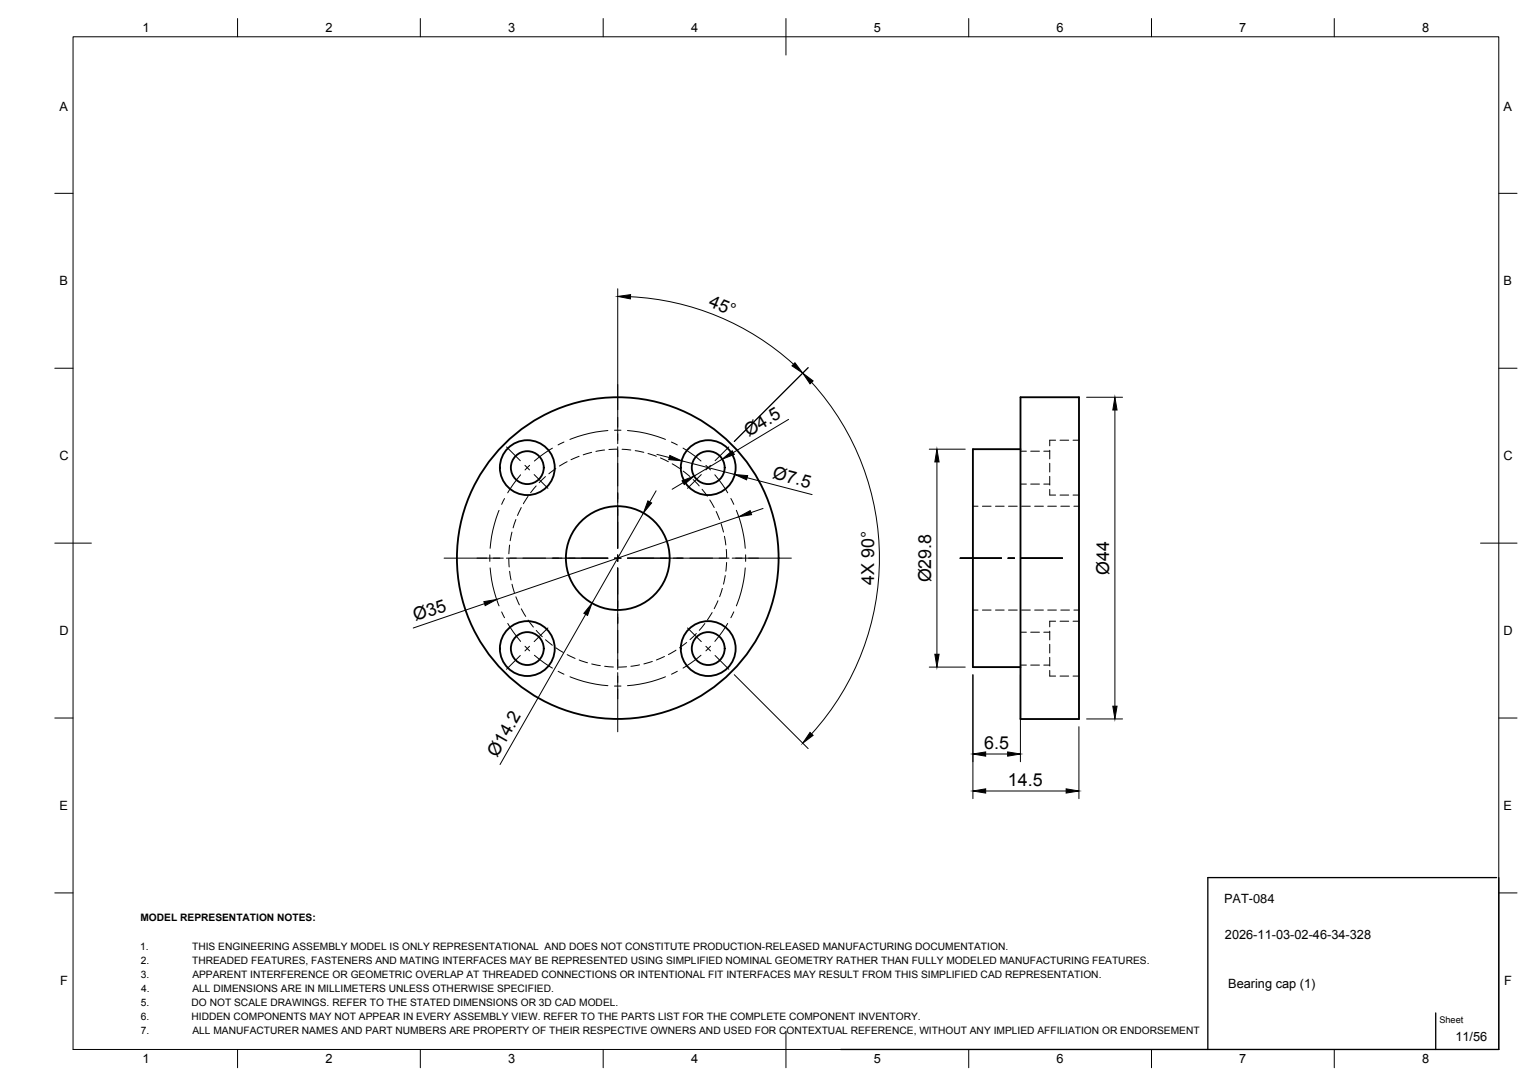
ISO-10303-21;
HEADER;
/* Generated by software containing ST-Developer
 * from STEP Tools, Inc. (www.steptools.com) 
 */

FILE_DESCRIPTION(
/* description */ ('Quick-return (Whitworth) mechanism'),
/* implementation_level */ '2;1');

FILE_NAME(
/* name */ 'Bearing cap (1).step',
/* time_stamp */ '2026-10-28T03:25:57-07:00',
/* author */ (''),
/* organization */ (''),
/* preprocessor_version */ 'ST-DEVELOPER v20.2',
/* originating_system */ 'Autodesk Translation Framework v15.17.0.0',
/* authorisation */ '');

FILE_SCHEMA (('AUTOMOTIVE_DESIGN { 1 0 10303 214 3 1 1 }'));
ENDSEC;

DATA;
#10=MECHANICAL_DESIGN_GEOMETRIC_PRESENTATION_REPRESENTATION('',(#496),#14878);
#408=SHAPE_REPRESENTATION_RELATIONSHIP('SRR','None',#15076,#452);
#452=ADVANCED_BREP_SHAPE_REPRESENTATION('',(#548),#14833);
#496=STYLED_ITEM('',(#15406),#548);
#548=MANIFOLD_SOLID_BREP('Body1',#7850);
#666=FACE_BOUND('',#1696,.T.);
#667=FACE_BOUND('',#1699,.T.);
#668=FACE_BOUND('',#1702,.T.);
#669=FACE_BOUND('',#1705,.T.);
#670=FACE_BOUND('',#1712,.T.);
#671=FACE_BOUND('',#1716,.T.);
#672=FACE_BOUND('',#1717,.T.);
#673=FACE_BOUND('',#1718,.T.);
#674=FACE_BOUND('',#1719,.T.);
#675=FACE_BOUND('',#1720,.T.);
#676=FACE_BOUND('',#1722,.T.);
#677=FACE_BOUND('',#1723,.T.);
#678=FACE_BOUND('',#1724,.T.);
#679=FACE_BOUND('',#1725,.T.);
#680=FACE_BOUND('',#1726,.T.);
#831=PLANE('',#8628);
#832=PLANE('',#8633);
#833=PLANE('',#8638);
#834=PLANE('',#8643);
#835=PLANE('',#8656);
#836=PLANE('',#8663);
#837=PLANE('',#8664);
#1153=FACE_OUTER_BOUND('',#1694,.T.);
#1154=FACE_OUTER_BOUND('',#1695,.T.);
#1155=FACE_OUTER_BOUND('',#1697,.T.);
#1156=FACE_OUTER_BOUND('',#1698,.T.);
#1157=FACE_OUTER_BOUND('',#1700,.T.);
#1158=FACE_OUTER_BOUND('',#1701,.T.);
#1159=FACE_OUTER_BOUND('',#1703,.T.);
#1160=FACE_OUTER_BOUND('',#1704,.T.);
#1161=FACE_OUTER_BOUND('',#1706,.T.);
#1162=FACE_OUTER_BOUND('',#1707,.T.);
#1163=FACE_OUTER_BOUND('',#1708,.T.);
#1164=FACE_OUTER_BOUND('',#1709,.T.);
#1165=FACE_OUTER_BOUND('',#1710,.T.);
#1166=FACE_OUTER_BOUND('',#1711,.T.);
#1167=FACE_OUTER_BOUND('',#1713,.T.);
#1168=FACE_OUTER_BOUND('',#1714,.T.);
#1169=FACE_OUTER_BOUND('',#1715,.T.);
#1170=FACE_OUTER_BOUND('',#1721,.T.);
#1694=EDGE_LOOP('',(#5732,#5733,#5734,#5735));
#1695=EDGE_LOOP('',(#5736));
#1696=EDGE_LOOP('',(#5737));
#1697=EDGE_LOOP('',(#5738,#5739,#5740,#5741));
#1698=EDGE_LOOP('',(#5742));
#1699=EDGE_LOOP('',(#5743));
#1700=EDGE_LOOP('',(#5744,#5745,#5746,#5747));
#1701=EDGE_LOOP('',(#5748));
#1702=EDGE_LOOP('',(#5749));
#1703=EDGE_LOOP('',(#5750,#5751,#5752,#5753));
#1704=EDGE_LOOP('',(#5754));
#1705=EDGE_LOOP('',(#5755));
#1706=EDGE_LOOP('',(#5756,#5757,#5758,#5759));
#1707=EDGE_LOOP('',(#5760,#5761,#5762,#5763));
#1708=EDGE_LOOP('',(#5764,#5765,#5766,#5767));
#1709=EDGE_LOOP('',(#5768,#5769,#5770,#5771));
#1710=EDGE_LOOP('',(#5772,#5773,#5774,#5775));
#1711=EDGE_LOOP('',(#5776));
#1712=EDGE_LOOP('',(#5777));
#1713=EDGE_LOOP('',(#5778,#5779,#5780,#5781));
#1714=EDGE_LOOP('',(#5782,#5783,#5784,#5785));
#1715=EDGE_LOOP('',(#5786));
#1716=EDGE_LOOP('',(#5787));
#1717=EDGE_LOOP('',(#5788));
#1718=EDGE_LOOP('',(#5789));
#1719=EDGE_LOOP('',(#5790));
#1720=EDGE_LOOP('',(#5791));
#1721=EDGE_LOOP('',(#5792));
#1722=EDGE_LOOP('',(#5793));
#1723=EDGE_LOOP('',(#5794));
#1724=EDGE_LOOP('',(#5795));
#1725=EDGE_LOOP('',(#5796));
#1726=EDGE_LOOP('',(#5797));
#2271=LINE('',#12594,#2794);
#2272=LINE('',#12603,#2795);
#2273=LINE('',#12612,#2796);
#2274=LINE('',#12621,#2797);
#2275=LINE('',#12629,#2798);
#2276=LINE('',#12633,#2799);
#2277=LINE('',#12637,#2800);
#2278=LINE('',#12641,#2801);
#2279=LINE('',#12646,#2802);
#2280=LINE('',#12654,#2803);
#2281=LINE('',#12659,#2804);
#2794=VECTOR('',#9984,0.375);
#2795=VECTOR('',#9995,0.375);
#2796=VECTOR('',#10006,0.375);
#2797=VECTOR('',#10017,0.375);
#2798=VECTOR('',#10028,0.225);
#2799=VECTOR('',#10033,0.225);
#2800=VECTOR('',#10038,0.225);
#2801=VECTOR('',#10043,0.225);
#2802=VECTOR('',#10048,1.49);
#2803=VECTOR('',#10059,0.71);
#2804=VECTOR('',#10064,2.2);
#3342=CIRCLE('',#8626,0.375);
#3343=CIRCLE('',#8627,0.375);
#3344=CIRCLE('',#8629,0.225);
#3345=CIRCLE('',#8631,0.375);
#3346=CIRCLE('',#8632,0.375);
#3347=CIRCLE('',#8634,0.225);
#3348=CIRCLE('',#8636,0.375);
#3349=CIRCLE('',#8637,0.375);
#3350=CIRCLE('',#8639,0.225);
#3351=CIRCLE('',#8641,0.375);
#3352=CIRCLE('',#8642,0.375);
#3353=CIRCLE('',#8644,0.225);
#3354=CIRCLE('',#8646,0.225);
#3355=CIRCLE('',#8648,0.225);
#3356=CIRCLE('',#8650,0.225);
#3357=CIRCLE('',#8652,0.225);
#3358=CIRCLE('',#8654,1.49);
#3359=CIRCLE('',#8655,1.49);
#3360=CIRCLE('',#8657,0.71);
#3361=CIRCLE('',#8659,0.71);
#3362=CIRCLE('',#8661,2.2);
#3363=CIRCLE('',#8662,2.2);
#3789=VERTEX_POINT('',#12591);
#3790=VERTEX_POINT('',#12593);
#3791=VERTEX_POINT('',#12597);
#3792=VERTEX_POINT('',#12600);
#3793=VERTEX_POINT('',#12602);
#3794=VERTEX_POINT('',#12606);
#3795=VERTEX_POINT('',#12609);
#3796=VERTEX_POINT('',#12611);
#3797=VERTEX_POINT('',#12615);
#3798=VERTEX_POINT('',#12618);
#3799=VERTEX_POINT('',#12620);
#3800=VERTEX_POINT('',#12624);
#3801=VERTEX_POINT('',#12627);
#3802=VERTEX_POINT('',#12631);
#3803=VERTEX_POINT('',#12635);
#3804=VERTEX_POINT('',#12639);
#3805=VERTEX_POINT('',#12643);
#3806=VERTEX_POINT('',#12645);
#3807=VERTEX_POINT('',#12649);
#3808=VERTEX_POINT('',#12652);
#3809=VERTEX_POINT('',#12656);
#3810=VERTEX_POINT('',#12658);
#4523=EDGE_CURVE('',#3789,#3789,#3342,.T.);
#4524=EDGE_CURVE('',#3789,#3790,#2271,.T.);
#4525=EDGE_CURVE('',#3790,#3790,#3343,.T.);
#4526=EDGE_CURVE('',#3791,#3791,#3344,.T.);
#4527=EDGE_CURVE('',#3792,#3792,#3345,.T.);
#4528=EDGE_CURVE('',#3792,#3793,#2272,.T.);
#4529=EDGE_CURVE('',#3793,#3793,#3346,.T.);
#4530=EDGE_CURVE('',#3794,#3794,#3347,.T.);
#4531=EDGE_CURVE('',#3795,#3795,#3348,.T.);
#4532=EDGE_CURVE('',#3795,#3796,#2273,.T.);
#4533=EDGE_CURVE('',#3796,#3796,#3349,.T.);
#4534=EDGE_CURVE('',#3797,#3797,#3350,.T.);
#4535=EDGE_CURVE('',#3798,#3798,#3351,.T.);
#4536=EDGE_CURVE('',#3798,#3799,#2274,.T.);
#4537=EDGE_CURVE('',#3799,#3799,#3352,.T.);
#4538=EDGE_CURVE('',#3800,#3800,#3353,.T.);
#4539=EDGE_CURVE('',#3801,#3801,#3354,.T.);
#4540=EDGE_CURVE('',#3801,#3791,#2275,.T.);
#4541=EDGE_CURVE('',#3802,#3802,#3355,.T.);
#4542=EDGE_CURVE('',#3802,#3794,#2276,.T.);
#4543=EDGE_CURVE('',#3803,#3803,#3356,.T.);
#4544=EDGE_CURVE('',#3803,#3797,#2277,.T.);
#4545=EDGE_CURVE('',#3804,#3804,#3357,.T.);
#4546=EDGE_CURVE('',#3804,#3800,#2278,.T.);
#4547=EDGE_CURVE('',#3805,#3805,#3358,.T.);
#4548=EDGE_CURVE('',#3805,#3806,#2279,.T.);
#4549=EDGE_CURVE('',#3806,#3806,#3359,.T.);
#4550=EDGE_CURVE('',#3807,#3807,#3360,.T.);
#4551=EDGE_CURVE('',#3808,#3808,#3361,.T.);
#4552=EDGE_CURVE('',#3808,#3807,#2280,.T.);
#4553=EDGE_CURVE('',#3809,#3809,#3362,.T.);
#4554=EDGE_CURVE('',#3809,#3810,#2281,.T.);
#4555=EDGE_CURVE('',#3810,#3810,#3363,.T.);
#5732=ORIENTED_EDGE('',*,*,#4523,.F.);
#5733=ORIENTED_EDGE('',*,*,#4524,.T.);
#5734=ORIENTED_EDGE('',*,*,#4525,.F.);
#5735=ORIENTED_EDGE('',*,*,#4524,.F.);
#5736=ORIENTED_EDGE('',*,*,#4523,.T.);
#5737=ORIENTED_EDGE('',*,*,#4526,.F.);
#5738=ORIENTED_EDGE('',*,*,#4527,.F.);
#5739=ORIENTED_EDGE('',*,*,#4528,.T.);
#5740=ORIENTED_EDGE('',*,*,#4529,.F.);
#5741=ORIENTED_EDGE('',*,*,#4528,.F.);
#5742=ORIENTED_EDGE('',*,*,#4527,.T.);
#5743=ORIENTED_EDGE('',*,*,#4530,.F.);
#5744=ORIENTED_EDGE('',*,*,#4531,.F.);
#5745=ORIENTED_EDGE('',*,*,#4532,.T.);
#5746=ORIENTED_EDGE('',*,*,#4533,.F.);
#5747=ORIENTED_EDGE('',*,*,#4532,.F.);
#5748=ORIENTED_EDGE('',*,*,#4531,.T.);
#5749=ORIENTED_EDGE('',*,*,#4534,.F.);
#5750=ORIENTED_EDGE('',*,*,#4535,.F.);
#5751=ORIENTED_EDGE('',*,*,#4536,.T.);
#5752=ORIENTED_EDGE('',*,*,#4537,.F.);
#5753=ORIENTED_EDGE('',*,*,#4536,.F.);
#5754=ORIENTED_EDGE('',*,*,#4535,.T.);
#5755=ORIENTED_EDGE('',*,*,#4538,.F.);
#5756=ORIENTED_EDGE('',*,*,#4539,.F.);
#5757=ORIENTED_EDGE('',*,*,#4540,.T.);
#5758=ORIENTED_EDGE('',*,*,#4526,.T.);
#5759=ORIENTED_EDGE('',*,*,#4540,.F.);
#5760=ORIENTED_EDGE('',*,*,#4541,.F.);
#5761=ORIENTED_EDGE('',*,*,#4542,.T.);
#5762=ORIENTED_EDGE('',*,*,#4530,.T.);
#5763=ORIENTED_EDGE('',*,*,#4542,.F.);
#5764=ORIENTED_EDGE('',*,*,#4543,.F.);
#5765=ORIENTED_EDGE('',*,*,#4544,.T.);
#5766=ORIENTED_EDGE('',*,*,#4534,.T.);
#5767=ORIENTED_EDGE('',*,*,#4544,.F.);
#5768=ORIENTED_EDGE('',*,*,#4545,.F.);
#5769=ORIENTED_EDGE('',*,*,#4546,.T.);
#5770=ORIENTED_EDGE('',*,*,#4538,.T.);
#5771=ORIENTED_EDGE('',*,*,#4546,.F.);
#5772=ORIENTED_EDGE('',*,*,#4547,.F.);
#5773=ORIENTED_EDGE('',*,*,#4548,.T.);
#5774=ORIENTED_EDGE('',*,*,#4549,.T.);
#5775=ORIENTED_EDGE('',*,*,#4548,.F.);
#5776=ORIENTED_EDGE('',*,*,#4549,.F.);
#5777=ORIENTED_EDGE('',*,*,#4550,.F.);
#5778=ORIENTED_EDGE('',*,*,#4551,.F.);
#5779=ORIENTED_EDGE('',*,*,#4552,.T.);
#5780=ORIENTED_EDGE('',*,*,#4550,.T.);
#5781=ORIENTED_EDGE('',*,*,#4552,.F.);
#5782=ORIENTED_EDGE('',*,*,#4553,.F.);
#5783=ORIENTED_EDGE('',*,*,#4554,.T.);
#5784=ORIENTED_EDGE('',*,*,#4555,.T.);
#5785=ORIENTED_EDGE('',*,*,#4554,.F.);
#5786=ORIENTED_EDGE('',*,*,#4553,.T.);
#5787=ORIENTED_EDGE('',*,*,#4551,.T.);
#5788=ORIENTED_EDGE('',*,*,#4537,.T.);
#5789=ORIENTED_EDGE('',*,*,#4533,.T.);
#5790=ORIENTED_EDGE('',*,*,#4529,.T.);
#5791=ORIENTED_EDGE('',*,*,#4525,.T.);
#5792=ORIENTED_EDGE('',*,*,#4555,.F.);
#5793=ORIENTED_EDGE('',*,*,#4547,.T.);
#5794=ORIENTED_EDGE('',*,*,#4545,.T.);
#5795=ORIENTED_EDGE('',*,*,#4543,.T.);
#5796=ORIENTED_EDGE('',*,*,#4541,.T.);
#5797=ORIENTED_EDGE('',*,*,#4539,.T.);
#7267=CYLINDRICAL_SURFACE('',#8625,0.375);
#7268=CYLINDRICAL_SURFACE('',#8630,0.375);
#7269=CYLINDRICAL_SURFACE('',#8635,0.375);
#7270=CYLINDRICAL_SURFACE('',#8640,0.375);
#7271=CYLINDRICAL_SURFACE('',#8645,0.225);
#7272=CYLINDRICAL_SURFACE('',#8647,0.225);
#7273=CYLINDRICAL_SURFACE('',#8649,0.225);
#7274=CYLINDRICAL_SURFACE('',#8651,0.225);
#7275=CYLINDRICAL_SURFACE('',#8653,1.49);
#7276=CYLINDRICAL_SURFACE('',#8658,0.71);
#7277=CYLINDRICAL_SURFACE('',#8660,2.2);
#7484=ADVANCED_FACE('',(#1153),#7267,.F.);
#7485=ADVANCED_FACE('',(#1154,#666),#831,.T.);
#7486=ADVANCED_FACE('',(#1155),#7268,.F.);
#7487=ADVANCED_FACE('',(#1156,#667),#832,.T.);
#7488=ADVANCED_FACE('',(#1157),#7269,.F.);
#7489=ADVANCED_FACE('',(#1158,#668),#833,.T.);
#7490=ADVANCED_FACE('',(#1159),#7270,.F.);
#7491=ADVANCED_FACE('',(#1160,#669),#834,.T.);
#7492=ADVANCED_FACE('',(#1161),#7271,.F.);
#7493=ADVANCED_FACE('',(#1162),#7272,.F.);
#7494=ADVANCED_FACE('',(#1163),#7273,.F.);
#7495=ADVANCED_FACE('',(#1164),#7274,.F.);
#7496=ADVANCED_FACE('',(#1165),#7275,.T.);
#7497=ADVANCED_FACE('',(#1166,#670),#835,.F.);
#7498=ADVANCED_FACE('',(#1167),#7276,.F.);
#7499=ADVANCED_FACE('',(#1168),#7277,.T.);
#7500=ADVANCED_FACE('',(#1169,#671,#672,#673,#674,#675),#836,.T.);
#7501=ADVANCED_FACE('',(#1170,#676,#677,#678,#679,#680),#837,.F.);
#7850=CLOSED_SHELL('',(#7484,#7485,#7486,#7487,#7488,#7489,#7490,#7491,
#7492,#7493,#7494,#7495,#7496,#7497,#7498,#7499,#7500,#7501));
#8624=AXIS2_PLACEMENT_3D('',#12589,#9978,#9979);
#8625=AXIS2_PLACEMENT_3D('',#12590,#9980,#9981);
#8626=AXIS2_PLACEMENT_3D('',#12592,#9982,#9983);
#8627=AXIS2_PLACEMENT_3D('',#12595,#9985,#9986);
#8628=AXIS2_PLACEMENT_3D('',#12596,#9987,#9988);
#8629=AXIS2_PLACEMENT_3D('',#12598,#9989,#9990);
#8630=AXIS2_PLACEMENT_3D('',#12599,#9991,#9992);
#8631=AXIS2_PLACEMENT_3D('',#12601,#9993,#9994);
#8632=AXIS2_PLACEMENT_3D('',#12604,#9996,#9997);
#8633=AXIS2_PLACEMENT_3D('',#12605,#9998,#9999);
#8634=AXIS2_PLACEMENT_3D('',#12607,#10000,#10001);
#8635=AXIS2_PLACEMENT_3D('',#12608,#10002,#10003);
#8636=AXIS2_PLACEMENT_3D('',#12610,#10004,#10005);
#8637=AXIS2_PLACEMENT_3D('',#12613,#10007,#10008);
#8638=AXIS2_PLACEMENT_3D('',#12614,#10009,#10010);
#8639=AXIS2_PLACEMENT_3D('',#12616,#10011,#10012);
#8640=AXIS2_PLACEMENT_3D('',#12617,#10013,#10014);
#8641=AXIS2_PLACEMENT_3D('',#12619,#10015,#10016);
#8642=AXIS2_PLACEMENT_3D('',#12622,#10018,#10019);
#8643=AXIS2_PLACEMENT_3D('',#12623,#10020,#10021);
#8644=AXIS2_PLACEMENT_3D('',#12625,#10022,#10023);
#8645=AXIS2_PLACEMENT_3D('',#12626,#10024,#10025);
#8646=AXIS2_PLACEMENT_3D('',#12628,#10026,#10027);
#8647=AXIS2_PLACEMENT_3D('',#12630,#10029,#10030);
#8648=AXIS2_PLACEMENT_3D('',#12632,#10031,#10032);
#8649=AXIS2_PLACEMENT_3D('',#12634,#10034,#10035);
#8650=AXIS2_PLACEMENT_3D('',#12636,#10036,#10037);
#8651=AXIS2_PLACEMENT_3D('',#12638,#10039,#10040);
#8652=AXIS2_PLACEMENT_3D('',#12640,#10041,#10042);
#8653=AXIS2_PLACEMENT_3D('',#12642,#10044,#10045);
#8654=AXIS2_PLACEMENT_3D('',#12644,#10046,#10047);
#8655=AXIS2_PLACEMENT_3D('',#12647,#10049,#10050);
#8656=AXIS2_PLACEMENT_3D('',#12648,#10051,#10052);
#8657=AXIS2_PLACEMENT_3D('',#12650,#10053,#10054);
#8658=AXIS2_PLACEMENT_3D('',#12651,#10055,#10056);
#8659=AXIS2_PLACEMENT_3D('',#12653,#10057,#10058);
#8660=AXIS2_PLACEMENT_3D('',#12655,#10060,#10061);
#8661=AXIS2_PLACEMENT_3D('',#12657,#10062,#10063);
#8662=AXIS2_PLACEMENT_3D('',#12660,#10065,#10066);
#8663=AXIS2_PLACEMENT_3D('',#12661,#10067,#10068);
#8664=AXIS2_PLACEMENT_3D('',#12662,#10069,#10070);
#9978=DIRECTION('axis',(0.,0.,1.));
#9979=DIRECTION('refdir',(1.,0.,0.));
#9980=DIRECTION('center_axis',(0.,0.,1.));
#9981=DIRECTION('ref_axis',(1.,0.,0.));
#9982=DIRECTION('center_axis',(0.,0.,1.));
#9983=DIRECTION('ref_axis',(1.,0.,0.));
#9984=DIRECTION('',(0.,0.,1.));
#9985=DIRECTION('center_axis',(0.,0.,-1.));
#9986=DIRECTION('ref_axis',(1.,0.,0.));
#9987=DIRECTION('center_axis',(0.,0.,1.));
#9988=DIRECTION('ref_axis',(1.,0.,0.));
#9989=DIRECTION('center_axis',(0.,0.,1.));
#9990=DIRECTION('ref_axis',(1.,0.,0.));
#9991=DIRECTION('center_axis',(0.,0.,1.));
#9992=DIRECTION('ref_axis',(1.,0.,0.));
#9993=DIRECTION('center_axis',(0.,0.,1.));
#9994=DIRECTION('ref_axis',(1.,0.,0.));
#9995=DIRECTION('',(0.,0.,1.));
#9996=DIRECTION('center_axis',(0.,0.,-1.));
#9997=DIRECTION('ref_axis',(1.,0.,0.));
#9998=DIRECTION('center_axis',(0.,0.,1.));
#9999=DIRECTION('ref_axis',(1.,0.,0.));
#10000=DIRECTION('center_axis',(0.,0.,1.));
#10001=DIRECTION('ref_axis',(1.,0.,0.));
#10002=DIRECTION('center_axis',(0.,0.,1.));
#10003=DIRECTION('ref_axis',(1.,0.,0.));
#10004=DIRECTION('center_axis',(0.,0.,1.));
#10005=DIRECTION('ref_axis',(1.,0.,0.));
#10006=DIRECTION('',(0.,0.,1.));
#10007=DIRECTION('center_axis',(0.,0.,-1.));
#10008=DIRECTION('ref_axis',(1.,0.,0.));
#10009=DIRECTION('center_axis',(0.,0.,1.));
#10010=DIRECTION('ref_axis',(1.,0.,0.));
#10011=DIRECTION('center_axis',(0.,0.,1.));
#10012=DIRECTION('ref_axis',(1.,0.,0.));
#10013=DIRECTION('center_axis',(0.,0.,1.));
#10014=DIRECTION('ref_axis',(1.,0.,0.));
#10015=DIRECTION('center_axis',(0.,0.,1.));
#10016=DIRECTION('ref_axis',(1.,0.,0.));
#10017=DIRECTION('',(0.,0.,1.));
#10018=DIRECTION('center_axis',(0.,0.,-1.));
#10019=DIRECTION('ref_axis',(1.,0.,0.));
#10020=DIRECTION('center_axis',(0.,0.,1.));
#10021=DIRECTION('ref_axis',(1.,0.,0.));
#10022=DIRECTION('center_axis',(0.,0.,1.));
#10023=DIRECTION('ref_axis',(1.,0.,0.));
#10024=DIRECTION('center_axis',(0.,0.,1.));
#10025=DIRECTION('ref_axis',(1.,0.,0.));
#10026=DIRECTION('center_axis',(0.,0.,1.));
#10027=DIRECTION('ref_axis',(1.,0.,0.));
#10028=DIRECTION('',(0.,0.,1.));
#10029=DIRECTION('center_axis',(0.,0.,1.));
#10030=DIRECTION('ref_axis',(1.,0.,0.));
#10031=DIRECTION('center_axis',(0.,0.,1.));
#10032=DIRECTION('ref_axis',(1.,0.,0.));
#10033=DIRECTION('',(0.,0.,1.));
#10034=DIRECTION('center_axis',(0.,0.,1.));
#10035=DIRECTION('ref_axis',(1.,0.,0.));
#10036=DIRECTION('center_axis',(0.,0.,1.));
#10037=DIRECTION('ref_axis',(1.,0.,0.));
#10038=DIRECTION('',(0.,0.,1.));
#10039=DIRECTION('center_axis',(0.,0.,1.));
#10040=DIRECTION('ref_axis',(1.,0.,0.));
#10041=DIRECTION('center_axis',(0.,0.,1.));
#10042=DIRECTION('ref_axis',(1.,0.,0.));
#10043=DIRECTION('',(0.,0.,1.));
#10044=DIRECTION('center_axis',(0.,0.,1.));
#10045=DIRECTION('ref_axis',(1.,0.,0.));
#10046=DIRECTION('center_axis',(0.,0.,1.));
#10047=DIRECTION('ref_axis',(1.,0.,0.));
#10048=DIRECTION('',(0.,0.,-1.));
#10049=DIRECTION('center_axis',(0.,0.,1.));
#10050=DIRECTION('ref_axis',(1.,0.,0.));
#10051=DIRECTION('center_axis',(0.,0.,1.));
#10052=DIRECTION('ref_axis',(1.,0.,0.));
#10053=DIRECTION('center_axis',(0.,0.,-1.));
#10054=DIRECTION('ref_axis',(1.,0.,0.));
#10055=DIRECTION('center_axis',(0.,0.,1.));
#10056=DIRECTION('ref_axis',(1.,0.,0.));
#10057=DIRECTION('center_axis',(0.,0.,-1.));
#10058=DIRECTION('ref_axis',(1.,0.,0.));
#10059=DIRECTION('',(0.,0.,-1.));
#10060=DIRECTION('center_axis',(0.,0.,1.));
#10061=DIRECTION('ref_axis',(1.,0.,0.));
#10062=DIRECTION('center_axis',(0.,0.,1.));
#10063=DIRECTION('ref_axis',(1.,0.,0.));
#10064=DIRECTION('',(0.,0.,-1.));
#10065=DIRECTION('center_axis',(0.,0.,1.));
#10066=DIRECTION('ref_axis',(1.,0.,0.));
#10067=DIRECTION('center_axis',(0.,0.,1.));
#10068=DIRECTION('ref_axis',(1.,0.,0.));
#10069=DIRECTION('center_axis',(0.,0.,1.));
#10070=DIRECTION('ref_axis',(1.,0.,0.));
#12589=CARTESIAN_POINT('',(0.,0.,0.));
#12590=CARTESIAN_POINT('Origin',(-1.23743686707646,4.76256313292354,4.));
#12591=CARTESIAN_POINT('',(-1.61243686707646,4.76256313292354,4.));
#12592=CARTESIAN_POINT('Origin',(-1.23743686707646,4.76256313292354,4.));
#12593=CARTESIAN_POINT('',(-1.61243686707646,4.76256313292354,4.4));
#12594=CARTESIAN_POINT('',(-1.61243686707646,4.76256313292354,4.));
#12595=CARTESIAN_POINT('Origin',(-1.23743686707646,4.76256313292354,4.4));
#12596=CARTESIAN_POINT('Origin',(-1.23743686707646,4.76256313292354,4.));
#12597=CARTESIAN_POINT('',(-1.46243686707646,4.76256313292354,4.));
#12598=CARTESIAN_POINT('Origin',(-1.23743686707646,4.76256313292354,4.));
#12599=CARTESIAN_POINT('Origin',(-1.23743686707646,7.23743686707646,4.));
#12600=CARTESIAN_POINT('',(-1.61243686707646,7.23743686707646,4.));
#12601=CARTESIAN_POINT('Origin',(-1.23743686707646,7.23743686707646,4.));
#12602=CARTESIAN_POINT('',(-1.61243686707646,7.23743686707646,4.4));
#12603=CARTESIAN_POINT('',(-1.61243686707646,7.23743686707646,4.));
#12604=CARTESIAN_POINT('Origin',(-1.23743686707646,7.23743686707646,4.4));
#12605=CARTESIAN_POINT('Origin',(-1.23743686707646,7.23743686707646,4.));
#12606=CARTESIAN_POINT('',(-1.46243686707646,7.23743686707646,4.));
#12607=CARTESIAN_POINT('Origin',(-1.23743686707646,7.23743686707646,4.));
#12608=CARTESIAN_POINT('Origin',(1.23743686707646,7.23743686707646,4.));
#12609=CARTESIAN_POINT('',(0.862436867076458,7.23743686707646,4.));
#12610=CARTESIAN_POINT('Origin',(1.23743686707646,7.23743686707646,4.));
#12611=CARTESIAN_POINT('',(0.862436867076458,7.23743686707646,4.4));
#12612=CARTESIAN_POINT('',(0.862436867076458,7.23743686707646,4.));
#12613=CARTESIAN_POINT('Origin',(1.23743686707646,7.23743686707646,4.4));
#12614=CARTESIAN_POINT('Origin',(1.23743686707646,7.23743686707646,4.));
#12615=CARTESIAN_POINT('',(1.01243686707646,7.23743686707646,4.));
#12616=CARTESIAN_POINT('Origin',(1.23743686707646,7.23743686707646,4.));
#12617=CARTESIAN_POINT('Origin',(1.23743686707646,4.76256313292354,4.));
#12618=CARTESIAN_POINT('',(0.862436867076458,4.76256313292354,4.));
#12619=CARTESIAN_POINT('Origin',(1.23743686707646,4.76256313292354,4.));
#12620=CARTESIAN_POINT('',(0.862436867076458,4.76256313292354,4.4));
#12621=CARTESIAN_POINT('',(0.862436867076458,4.76256313292354,4.));
#12622=CARTESIAN_POINT('Origin',(1.23743686707646,4.76256313292354,4.4));
#12623=CARTESIAN_POINT('Origin',(1.23743686707646,4.76256313292354,4.));
#12624=CARTESIAN_POINT('',(1.01243686707646,4.76256313292354,4.));
#12625=CARTESIAN_POINT('Origin',(1.23743686707646,4.76256313292354,4.));
#12626=CARTESIAN_POINT('Origin',(-1.23743686707646,4.76256313292354,3.5));
#12627=CARTESIAN_POINT('',(-1.46243686707646,4.76256313292354,3.6));
#12628=CARTESIAN_POINT('Origin',(-1.23743686707646,4.76256313292354,3.6));
#12629=CARTESIAN_POINT('',(-1.46243686707646,4.76256313292354,3.5));
#12630=CARTESIAN_POINT('Origin',(-1.23743686707646,7.23743686707646,3.5));
#12631=CARTESIAN_POINT('',(-1.46243686707646,7.23743686707646,3.6));
#12632=CARTESIAN_POINT('Origin',(-1.23743686707646,7.23743686707646,3.6));
#12633=CARTESIAN_POINT('',(-1.46243686707646,7.23743686707646,3.5));
#12634=CARTESIAN_POINT('Origin',(1.23743686707646,7.23743686707646,3.5));
#12635=CARTESIAN_POINT('',(1.01243686707646,7.23743686707646,3.6));
#12636=CARTESIAN_POINT('Origin',(1.23743686707646,7.23743686707646,3.6));
#12637=CARTESIAN_POINT('',(1.01243686707646,7.23743686707646,3.5));
#12638=CARTESIAN_POINT('Origin',(1.23743686707646,4.76256313292354,3.5));
#12639=CARTESIAN_POINT('',(1.01243686707646,4.76256313292354,3.6));
#12640=CARTESIAN_POINT('Origin',(1.23743686707646,4.76256313292354,3.6));
#12641=CARTESIAN_POINT('',(1.01243686707646,4.76256313292354,3.5));
#12642=CARTESIAN_POINT('Origin',(0.,6.,2.95));
#12643=CARTESIAN_POINT('',(-1.49,6.,3.6));
#12644=CARTESIAN_POINT('Origin',(0.,6.,3.6));
#12645=CARTESIAN_POINT('',(-1.49,6.,2.95));
#12646=CARTESIAN_POINT('',(-1.49,6.,2.95));
#12647=CARTESIAN_POINT('Origin',(0.,6.,2.95));
#12648=CARTESIAN_POINT('Origin',(0.,6.,2.95));
#12649=CARTESIAN_POINT('',(-0.71,6.,2.95));
#12650=CARTESIAN_POINT('Origin',(0.,6.,2.95));
#12651=CARTESIAN_POINT('Origin',(0.,6.,3.6));
#12652=CARTESIAN_POINT('',(-0.71,6.,4.4));
#12653=CARTESIAN_POINT('Origin',(0.,6.,4.4));
#12654=CARTESIAN_POINT('',(-0.71,6.,3.6));
#12655=CARTESIAN_POINT('Origin',(0.,6.,3.6));
#12656=CARTESIAN_POINT('',(-2.2,6.,4.4));
#12657=CARTESIAN_POINT('Origin',(0.,6.,4.4));
#12658=CARTESIAN_POINT('',(-2.2,6.,3.6));
#12659=CARTESIAN_POINT('',(-2.2,6.,3.6));
#12660=CARTESIAN_POINT('Origin',(0.,6.,3.6));
#12661=CARTESIAN_POINT('Origin',(0.,6.,4.4));
#12662=CARTESIAN_POINT('Origin',(0.,6.,3.6));
#14779=UNCERTAINTY_MEASURE_WITH_UNIT(LENGTH_MEASURE(0.001),#14879,
'DISTANCE_ACCURACY_VALUE',
'Maximum model space distance between geometric entities at asserted c
onnectivities');
#14824=UNCERTAINTY_MEASURE_WITH_UNIT(LENGTH_MEASURE(0.001),#14879,
'DISTANCE_ACCURACY_VALUE',
'Maximum model space distance between geometric entities at asserted c
onnectivities');
#14833=(
GEOMETRIC_REPRESENTATION_CONTEXT(3)
GLOBAL_UNCERTAINTY_ASSIGNED_CONTEXT((#14779))
GLOBAL_UNIT_ASSIGNED_CONTEXT((#14879,#14881,#14882))
REPRESENTATION_CONTEXT('','3D')
);
#14878=(
GEOMETRIC_REPRESENTATION_CONTEXT(3)
GLOBAL_UNCERTAINTY_ASSIGNED_CONTEXT((#14824))
GLOBAL_UNIT_ASSIGNED_CONTEXT((#14879,#14881,#14882))
REPRESENTATION_CONTEXT('','3D')
);
#14879=(
LENGTH_UNIT()
NAMED_UNIT(*)
SI_UNIT(.CENTI.,.METRE.)
);
#14881=(
NAMED_UNIT(*)
PLANE_ANGLE_UNIT()
SI_UNIT($,.RADIAN.)
);
#14882=(
NAMED_UNIT(*)
SI_UNIT($,.STERADIAN.)
SOLID_ANGLE_UNIT()
);
#14891=SHAPE_DEFINITION_REPRESENTATION(#14944,#15076);
#14944=PRODUCT_DEFINITION_SHAPE('',$,#15130);
#15076=SHAPE_REPRESENTATION('',(#8624),#14833);
#15121=PRODUCT_DEFINITION_CONTEXT('part definition',#15282,'design');
#15130=PRODUCT_DEFINITION('Bearing cap (1)','Bearing cap (1)',#15183,#15121);
#15183=PRODUCT_DEFINITION_FORMATION('',$,#15292);
#15282=APPLICATION_CONTEXT(
'Core Data for Automotive Mechanical Design Process');
#15283=PRODUCT_CONTEXT('part definition',#15282,'mechanical');
#15292=PRODUCT('Bearing cap (1)','Bearing cap (1)','Bearing cap (1)',(#15283));
#15400=COLOUR_RGB('Grey',0.48,0.52,0.57);
#15401=FILL_AREA_STYLE_COLOUR('',#15400);
#15402=FILL_AREA_STYLE('',(#15401));
#15403=SURFACE_STYLE_FILL_AREA(#15402);
#15404=SURFACE_SIDE_STYLE('',(#15403));
#15405=SURFACE_STYLE_USAGE(.BOTH.,#15404);
#15406=PRESENTATION_STYLE_ASSIGNMENT((#15405));
ENDSEC;
END-ISO-10303-21;
